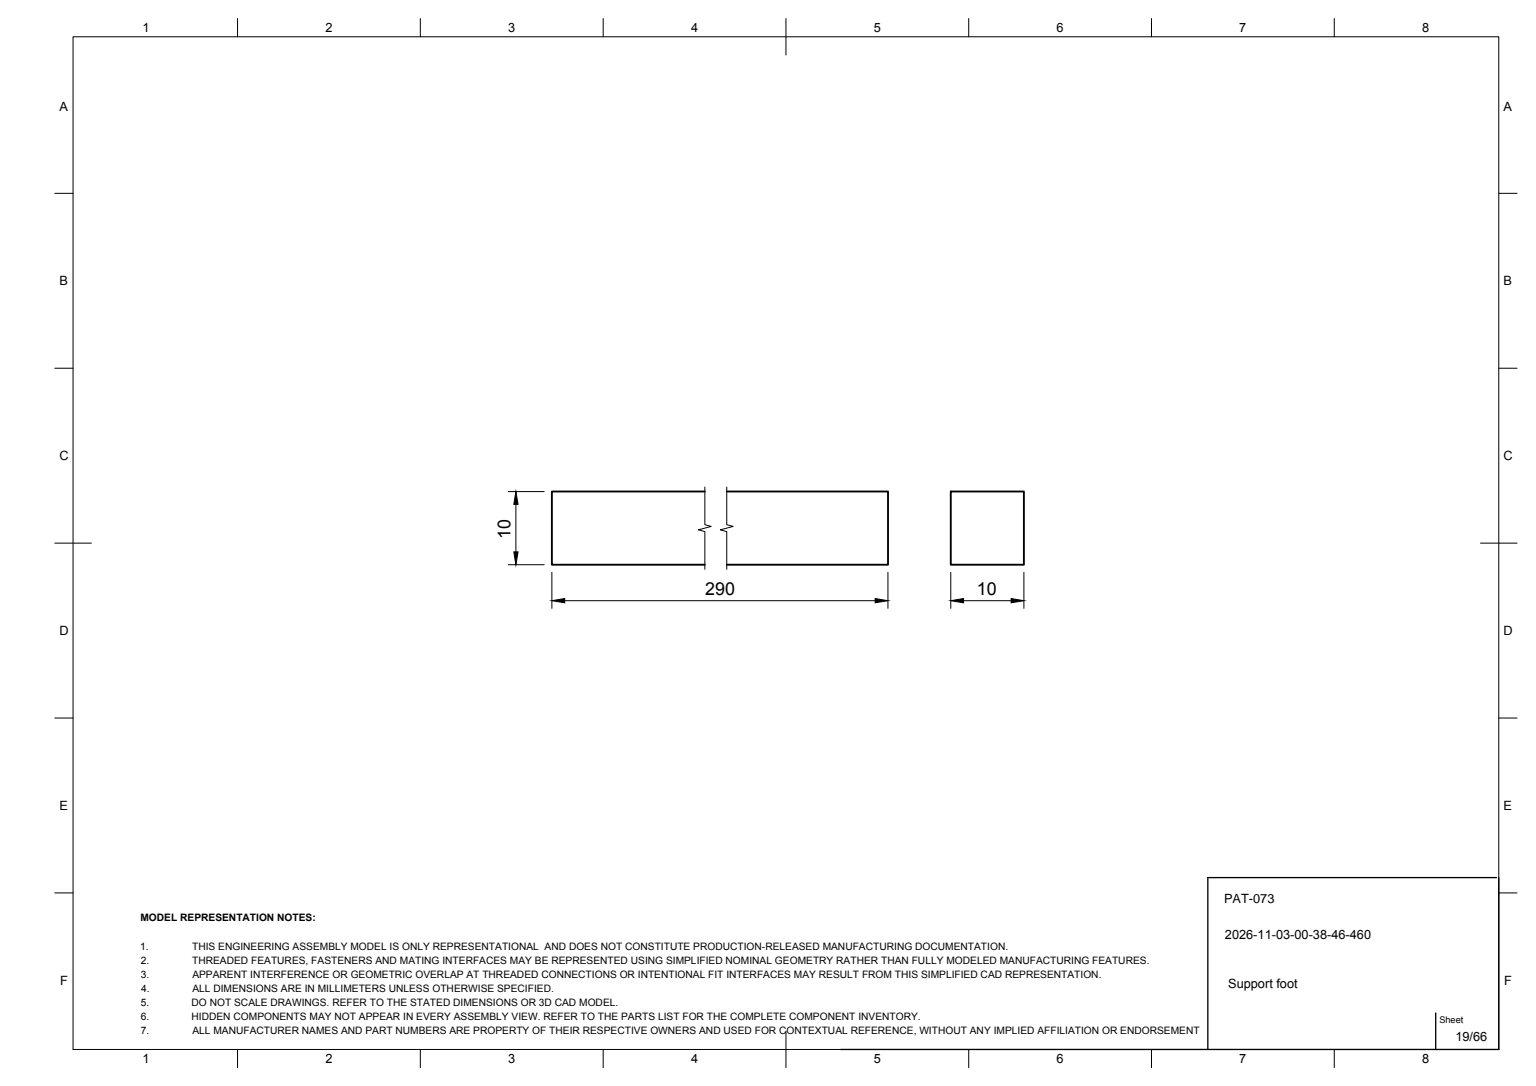
ISO-10303-21;
HEADER;
/* Generated by software containing ST-Developer
 * from STEP Tools, Inc. (www.steptools.com) 
 */

FILE_DESCRIPTION(
/* description */ ('Manual piston pump'),
/* implementation_level */ '2;1');

FILE_NAME(
/* name */ 'Support foot.step',
/* time_stamp */ '2026-11-02T16:54:23-08:00',
/* author */ (''),
/* organization */ (''),
/* preprocessor_version */ 'ST-DEVELOPER v20.2',
/* originating_system */ 'Autodesk Translation Framework v15.17.0.0',
/* authorisation */ '');

FILE_SCHEMA (('AUTOMOTIVE_DESIGN { 1 0 10303 214 3 1 1 }'));
ENDSEC;

DATA;
#10=MECHANICAL_DESIGN_GEOMETRIC_PRESENTATION_REPRESENTATION('',(#705),#19043);
#579=SHAPE_REPRESENTATION_RELATIONSHIP('SRR','None',#19325,#642);
#642=ADVANCED_BREP_SHAPE_REPRESENTATION('',(#776),#18992);
#705=STYLED_ITEM('',(#19662),#776);
#776=MANIFOLD_SOLID_BREP('Body1',#9490);
#1456=FACE_OUTER_BOUND('',#2105,.T.);
#1457=FACE_OUTER_BOUND('',#2106,.T.);
#1458=FACE_OUTER_BOUND('',#2107,.T.);
#1459=FACE_OUTER_BOUND('',#2108,.T.);
#1460=FACE_OUTER_BOUND('',#2109,.T.);
#1461=FACE_OUTER_BOUND('',#2110,.T.);
#2105=EDGE_LOOP('',(#6937,#6938,#6939,#6940));
#2106=EDGE_LOOP('',(#6941,#6942,#6943,#6944));
#2107=EDGE_LOOP('',(#6945,#6946,#6947,#6948));
#2108=EDGE_LOOP('',(#6949,#6950,#6951,#6952));
#2109=EDGE_LOOP('',(#6953,#6954,#6955,#6956));
#2110=EDGE_LOOP('',(#6957,#6958,#6959,#6960));
#3325=LINE('',#15415,#3929);
#3326=LINE('',#15417,#3930);
#3327=LINE('',#15419,#3931);
#3328=LINE('',#15420,#3932);
#3329=LINE('',#15423,#3933);
#3330=LINE('',#15425,#3934);
#3331=LINE('',#15426,#3935);
#3332=LINE('',#15429,#3936);
#3333=LINE('',#15431,#3937);
#3334=LINE('',#15432,#3938);
#3335=LINE('',#15434,#3939);
#3336=LINE('',#15435,#3940);
#3929=VECTOR('',#12321,1.);
#3930=VECTOR('',#12322,1.);
#3931=VECTOR('',#12323,1.);
#3932=VECTOR('',#12324,1.);
#3933=VECTOR('',#12327,1.);
#3934=VECTOR('',#12328,1.);
#3935=VECTOR('',#12329,1.);
#3936=VECTOR('',#12332,1.);
#3937=VECTOR('',#12333,1.);
#3938=VECTOR('',#12334,1.);
#3939=VECTOR('',#12337,1.);
#3940=VECTOR('',#12338,1.);
#4573=VERTEX_POINT('',#15413);
#4574=VERTEX_POINT('',#15414);
#4575=VERTEX_POINT('',#15416);
#4576=VERTEX_POINT('',#15418);
#4577=VERTEX_POINT('',#15422);
#4578=VERTEX_POINT('',#15424);
#4579=VERTEX_POINT('',#15428);
#4580=VERTEX_POINT('',#15430);
#5455=EDGE_CURVE('',#4573,#4574,#3325,.T.);
#5456=EDGE_CURVE('',#4574,#4575,#3326,.T.);
#5457=EDGE_CURVE('',#4576,#4575,#3327,.T.);
#5458=EDGE_CURVE('',#4573,#4576,#3328,.T.);
#5459=EDGE_CURVE('',#4577,#4573,#3329,.T.);
#5460=EDGE_CURVE('',#4578,#4576,#3330,.T.);
#5461=EDGE_CURVE('',#4577,#4578,#3331,.T.);
#5462=EDGE_CURVE('',#4579,#4577,#3332,.T.);
#5463=EDGE_CURVE('',#4580,#4578,#3333,.T.);
#5464=EDGE_CURVE('',#4579,#4580,#3334,.T.);
#5465=EDGE_CURVE('',#4574,#4579,#3335,.T.);
#5466=EDGE_CURVE('',#4575,#4580,#3336,.T.);
#6937=ORIENTED_EDGE('',*,*,#5455,.T.);
#6938=ORIENTED_EDGE('',*,*,#5456,.T.);
#6939=ORIENTED_EDGE('',*,*,#5457,.F.);
#6940=ORIENTED_EDGE('',*,*,#5458,.F.);
#6941=ORIENTED_EDGE('',*,*,#5459,.T.);
#6942=ORIENTED_EDGE('',*,*,#5458,.T.);
#6943=ORIENTED_EDGE('',*,*,#5460,.F.);
#6944=ORIENTED_EDGE('',*,*,#5461,.F.);
#6945=ORIENTED_EDGE('',*,*,#5462,.T.);
#6946=ORIENTED_EDGE('',*,*,#5461,.T.);
#6947=ORIENTED_EDGE('',*,*,#5463,.F.);
#6948=ORIENTED_EDGE('',*,*,#5464,.F.);
#6949=ORIENTED_EDGE('',*,*,#5465,.T.);
#6950=ORIENTED_EDGE('',*,*,#5464,.T.);
#6951=ORIENTED_EDGE('',*,*,#5466,.F.);
#6952=ORIENTED_EDGE('',*,*,#5456,.F.);
#6953=ORIENTED_EDGE('',*,*,#5466,.T.);
#6954=ORIENTED_EDGE('',*,*,#5463,.T.);
#6955=ORIENTED_EDGE('',*,*,#5460,.T.);
#6956=ORIENTED_EDGE('',*,*,#5457,.T.);
#6957=ORIENTED_EDGE('',*,*,#5465,.F.);
#6958=ORIENTED_EDGE('',*,*,#5455,.F.);
#6959=ORIENTED_EDGE('',*,*,#5459,.F.);
#6960=ORIENTED_EDGE('',*,*,#5462,.F.);
#8665=PLANE('',#10566);
#8666=PLANE('',#10567);
#8667=PLANE('',#10568);
#8668=PLANE('',#10569);
#8669=PLANE('',#10570);
#8670=PLANE('',#10571);
#9061=ADVANCED_FACE('',(#1456),#8665,.T.);
#9062=ADVANCED_FACE('',(#1457),#8666,.T.);
#9063=ADVANCED_FACE('',(#1458),#8667,.T.);
#9064=ADVANCED_FACE('',(#1459),#8668,.T.);
#9065=ADVANCED_FACE('',(#1460),#8669,.T.);
#9066=ADVANCED_FACE('',(#1461),#8670,.F.);
#9490=CLOSED_SHELL('',(#9061,#9062,#9063,#9064,#9065,#9066));
#10565=AXIS2_PLACEMENT_3D('',#15411,#12317,#12318);
#10566=AXIS2_PLACEMENT_3D('',#15412,#12319,#12320);
#10567=AXIS2_PLACEMENT_3D('',#15421,#12325,#12326);
#10568=AXIS2_PLACEMENT_3D('',#15427,#12330,#12331);
#10569=AXIS2_PLACEMENT_3D('',#15433,#12335,#12336);
#10570=AXIS2_PLACEMENT_3D('',#15436,#12339,#12340);
#10571=AXIS2_PLACEMENT_3D('',#15437,#12341,#12342);
#12317=DIRECTION('axis',(0.,0.,1.));
#12318=DIRECTION('refdir',(1.,0.,0.));
#12319=DIRECTION('center_axis',(0.,1.,0.));
#12320=DIRECTION('ref_axis',(-1.,0.,0.));
#12321=DIRECTION('',(-1.,0.,0.));
#12322=DIRECTION('',(0.,0.,1.));
#12323=DIRECTION('',(-1.,0.,0.));
#12324=DIRECTION('',(0.,0.,1.));
#12325=DIRECTION('center_axis',(1.,0.,0.));
#12326=DIRECTION('ref_axis',(0.,1.,0.));
#12327=DIRECTION('',(0.,1.,0.));
#12328=DIRECTION('',(0.,1.,0.));
#12329=DIRECTION('',(0.,0.,1.));
#12330=DIRECTION('center_axis',(0.,-1.,0.));
#12331=DIRECTION('ref_axis',(1.,0.,0.));
#12332=DIRECTION('',(1.,0.,0.));
#12333=DIRECTION('',(1.,0.,0.));
#12334=DIRECTION('',(0.,0.,1.));
#12335=DIRECTION('center_axis',(-1.,0.,0.));
#12336=DIRECTION('ref_axis',(0.,-1.,0.));
#12337=DIRECTION('',(0.,-1.,0.));
#12338=DIRECTION('',(0.,-1.,0.));
#12339=DIRECTION('center_axis',(0.,0.,1.));
#12340=DIRECTION('ref_axis',(1.,0.,0.));
#12341=DIRECTION('center_axis',(0.,0.,1.));
#12342=DIRECTION('ref_axis',(1.,0.,0.));
#15411=CARTESIAN_POINT('',(0.,0.,0.));
#15412=CARTESIAN_POINT('Origin',(-3.5,15.,-2.));
#15413=CARTESIAN_POINT('',(-3.5,15.,-2.));
#15414=CARTESIAN_POINT('',(-4.5,15.,-2.));
#15415=CARTESIAN_POINT('',(-3.5,15.,-2.));
#15416=CARTESIAN_POINT('',(-4.5,15.,-1.));
#15417=CARTESIAN_POINT('',(-4.5,15.,-2.));
#15418=CARTESIAN_POINT('',(-3.5,15.,-1.));
#15419=CARTESIAN_POINT('',(-3.5,15.,-1.));
#15420=CARTESIAN_POINT('',(-3.5,15.,-2.));
#15421=CARTESIAN_POINT('Origin',(-3.5,-14.,-2.));
#15422=CARTESIAN_POINT('',(-3.5,-14.,-2.));
#15423=CARTESIAN_POINT('',(-3.5,-14.,-2.));
#15424=CARTESIAN_POINT('',(-3.5,-14.,-1.));
#15425=CARTESIAN_POINT('',(-3.5,-14.,-1.));
#15426=CARTESIAN_POINT('',(-3.5,-14.,-2.));
#15427=CARTESIAN_POINT('Origin',(-4.5,-14.,-2.));
#15428=CARTESIAN_POINT('',(-4.5,-14.,-2.));
#15429=CARTESIAN_POINT('',(-4.5,-14.,-2.));
#15430=CARTESIAN_POINT('',(-4.5,-14.,-1.));
#15431=CARTESIAN_POINT('',(-4.5,-14.,-1.));
#15432=CARTESIAN_POINT('',(-4.5,-14.,-2.));
#15433=CARTESIAN_POINT('Origin',(-4.5,15.,-2.));
#15434=CARTESIAN_POINT('',(-4.5,15.,-2.));
#15435=CARTESIAN_POINT('',(-4.5,15.,-1.));
#15436=CARTESIAN_POINT('Origin',(-4.,0.5,-1.));
#15437=CARTESIAN_POINT('Origin',(-4.,0.5,-2.));
#18921=UNCERTAINTY_MEASURE_WITH_UNIT(LENGTH_MEASURE(0.001),#19044,
'DISTANCE_ACCURACY_VALUE',
'Maximum model space distance between geometric entities at asserted c
onnectivities');
#18972=UNCERTAINTY_MEASURE_WITH_UNIT(LENGTH_MEASURE(0.001),#19044,
'DISTANCE_ACCURACY_VALUE',
'Maximum model space distance between geometric entities at asserted c
onnectivities');
#18992=(
GEOMETRIC_REPRESENTATION_CONTEXT(3)
GLOBAL_UNCERTAINTY_ASSIGNED_CONTEXT((#18921))
GLOBAL_UNIT_ASSIGNED_CONTEXT((#19044,#19046,#19047))
REPRESENTATION_CONTEXT('','3D')
);
#19043=(
GEOMETRIC_REPRESENTATION_CONTEXT(3)
GLOBAL_UNCERTAINTY_ASSIGNED_CONTEXT((#18972))
GLOBAL_UNIT_ASSIGNED_CONTEXT((#19044,#19046,#19047))
REPRESENTATION_CONTEXT('','3D')
);
#19044=(
LENGTH_UNIT()
NAMED_UNIT(*)
SI_UNIT(.CENTI.,.METRE.)
);
#19046=(
NAMED_UNIT(*)
PLANE_ANGLE_UNIT()
SI_UNIT($,.RADIAN.)
);
#19047=(
NAMED_UNIT(*)
SI_UNIT($,.STERADIAN.)
SOLID_ANGLE_UNIT()
);
#19067=SHAPE_DEFINITION_REPRESENTATION(#19137,#19325);
#19137=PRODUCT_DEFINITION_SHAPE('',$,#19396);
#19325=SHAPE_REPRESENTATION('',(#10565),#18992);
#19376=PRODUCT_DEFINITION_CONTEXT('part definition',#19588,'design');
#19396=PRODUCT_DEFINITION('2026-11-03-00-38-46-460','Support foot',#19466,
#19376);
#19466=PRODUCT_DEFINITION_FORMATION('',$,#19609);
#19588=APPLICATION_CONTEXT(
'Core Data for Automotive Mechanical Design Process');
#19589=PRODUCT_CONTEXT('part definition',#19588,'mechanical');
#19609=PRODUCT('2026-11-03-00-38-46-460','Support foot','Support foot',
(#19589));
#19662=PRESENTATION_STYLE_ASSIGNMENT((#19668));
#19668=SURFACE_STYLE_USAGE(.BOTH.,#19674);
#19674=SURFACE_SIDE_STYLE('',(#19680));
#19680=SURFACE_STYLE_FILL_AREA(#19686);
#19686=FILL_AREA_STYLE('CAD Library Painted - Deep blue',(#19692));
#19692=FILL_AREA_STYLE_COLOUR('CAD Library Painted - Deep blue',#19698);
#19698=COLOUR_RGB('CAD Library Painted - Deep blue',0.0784313725490196,
0.203921568627451,0.349019607843137);
ENDSEC;
END-ISO-10303-21;
